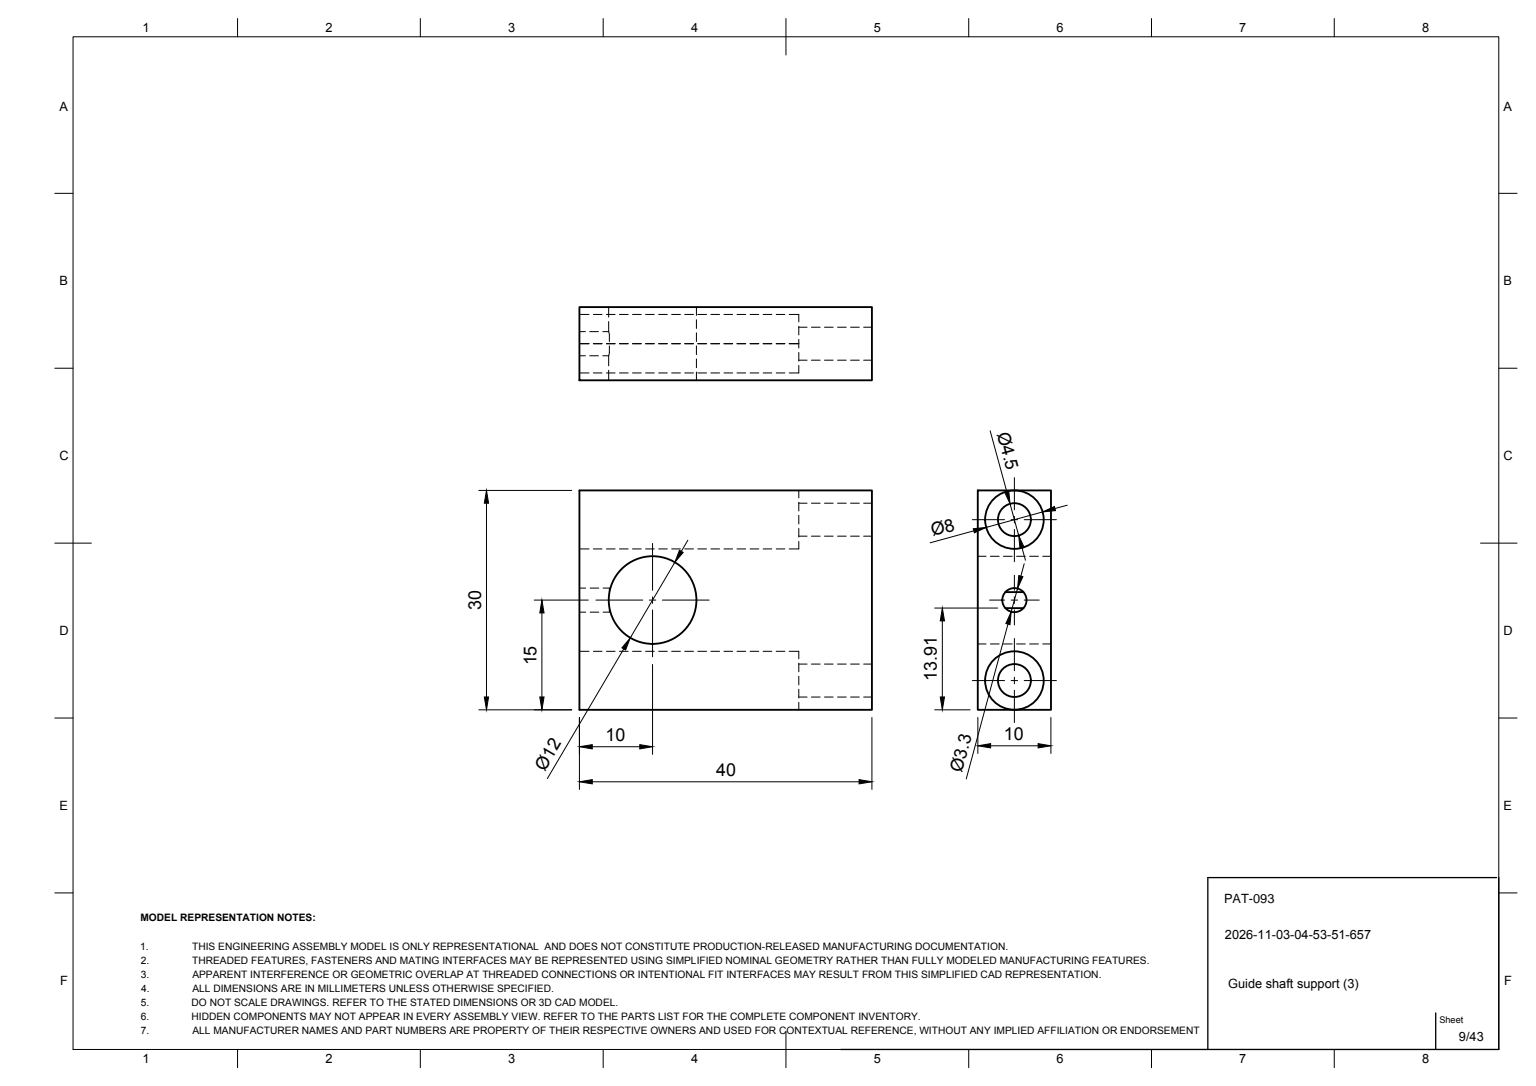
ISO-10303-21;
HEADER;
/* Generated by software containing ST-Developer
 * from STEP Tools, Inc. (www.steptools.com) 
 */

FILE_DESCRIPTION(
/* description */ ('Self-centering screw clamp'),
/* implementation_level */ '2;1');

FILE_NAME(
/* name */ 'Guide shaft support (3).step',
/* time_stamp */ '2026-10-28T03:25:31-07:00',
/* author */ (''),
/* organization */ (''),
/* preprocessor_version */ 'ST-DEVELOPER v20.2',
/* originating_system */ 'Autodesk Translation Framework v15.17.0.0',
/* authorisation */ '');

FILE_SCHEMA (('AUTOMOTIVE_DESIGN { 1 0 10303 214 3 1 1 }'));
ENDSEC;

DATA;
#10=MECHANICAL_DESIGN_GEOMETRIC_PRESENTATION_REPRESENTATION('',(#630),#16799);
#510=B_SPLINE_CURVE_WITH_KNOTS('',3,(#14205,#14206,#14207,#14208,#14209,
#14210),.UNSPECIFIED.,.F.,.F.,(4,2,4),(0.635430324955931,0.687528937234027,
0.750024497760672),.UNSPECIFIED.);
#511=B_SPLINE_CURVE_WITH_KNOTS('',3,(#14214,#14215,#14216,#14217,#14218,
#14219),.UNSPECIFIED.,.F.,.F.,(4,2,4),(0.250008165920224,0.312503726446869,
0.364602338724964),.UNSPECIFIED.);
#512=B_SPLINE_CURVE_WITH_KNOTS('',3,(#14220,#14221,#14222,#14223,#14224,
#14225),.UNSPECIFIED.,.F.,.F.,(4,2,4),(0.135413993115483,0.187512605393579,
0.250008165920224),.UNSPECIFIED.);
#513=B_SPLINE_CURVE_WITH_KNOTS('',3,(#14226,#14227,#14228,#14229,#14230,
#14231),.UNSPECIFIED.,.F.,.F.,(4,2,4),(0.750024497760672,0.812520058287317,
0.864618670565414),.UNSPECIFIED.);
#548=SHAPE_REPRESENTATION_RELATIONSHIP('SRR','None',#17021,#589);
#589=ADVANCED_BREP_SHAPE_REPRESENTATION('',(#678),#16759);
#630=STYLED_ITEM('',(#17326),#678);
#678=MANIFOLD_SOLID_BREP('Body1',#9081);
#763=FACE_BOUND('',#1913,.T.);
#764=FACE_BOUND('',#1916,.T.);
#765=FACE_BOUND('',#1918,.T.);
#766=FACE_BOUND('',#1924,.T.);
#767=FACE_BOUND('',#1927,.T.);
#768=FACE_BOUND('',#1929,.T.);
#769=FACE_BOUND('',#1930,.T.);
#1062=PLANE('',#9751);
#1063=PLANE('',#9756);
#1064=PLANE('',#9760);
#1065=PLANE('',#9765);
#1066=PLANE('',#9767);
#1067=PLANE('',#9775);
#1068=PLANE('',#9776);
#1069=PLANE('',#9777);
#1070=PLANE('',#9778);
#1071=PLANE('',#9779);
#1357=FACE_OUTER_BOUND('',#1906,.T.);
#1358=FACE_OUTER_BOUND('',#1907,.T.);
#1359=FACE_OUTER_BOUND('',#1908,.T.);
#1360=FACE_OUTER_BOUND('',#1909,.T.);
#1361=FACE_OUTER_BOUND('',#1910,.T.);
#1362=FACE_OUTER_BOUND('',#1911,.T.);
#1363=FACE_OUTER_BOUND('',#1912,.T.);
#1364=FACE_OUTER_BOUND('',#1914,.T.);
#1365=FACE_OUTER_BOUND('',#1915,.T.);
#1366=FACE_OUTER_BOUND('',#1917,.T.);
#1367=FACE_OUTER_BOUND('',#1919,.T.);
#1368=FACE_OUTER_BOUND('',#1920,.T.);
#1369=FACE_OUTER_BOUND('',#1921,.T.);
#1370=FACE_OUTER_BOUND('',#1922,.T.);
#1371=FACE_OUTER_BOUND('',#1923,.T.);
#1372=FACE_OUTER_BOUND('',#1925,.T.);
#1373=FACE_OUTER_BOUND('',#1926,.T.);
#1374=FACE_OUTER_BOUND('',#1928,.T.);
#1906=EDGE_LOOP('',(#6535,#6536,#6537,#6538));
#1907=EDGE_LOOP('',(#6539,#6540,#6541,#6542));
#1908=EDGE_LOOP('',(#6543,#6544));
#1909=EDGE_LOOP('',(#6545,#6546,#6547,#6548,#6549,#6550,#6551,#6552,#6553));
#1910=EDGE_LOOP('',(#6554,#6555));
#1911=EDGE_LOOP('',(#6556,#6557,#6558,#6559));
#1912=EDGE_LOOP('',(#6560,#6561));
#1913=EDGE_LOOP('',(#6562));
#1914=EDGE_LOOP('',(#6563,#6564,#6565,#6566));
#1915=EDGE_LOOP('',(#6567,#6568));
#1916=EDGE_LOOP('',(#6569));
#1917=EDGE_LOOP('',(#6570,#6571,#6572,#6573,#6574,#6575,#6576,#6577,#6578,
#6579));
#1918=EDGE_LOOP('',(#6580));
#1919=EDGE_LOOP('',(#6581,#6582,#6583,#6584));
#1920=EDGE_LOOP('',(#6585,#6586,#6587,#6588));
#1921=EDGE_LOOP('',(#6589,#6590,#6591,#6592,#6593,#6594,#6595,#6596,#6597,
#6598,#6599,#6600));
#1922=EDGE_LOOP('',(#6601,#6602,#6603,#6604,#6605,#6606,#6607));
#1923=EDGE_LOOP('',(#6608,#6609,#6610,#6611));
#1924=EDGE_LOOP('',(#6612));
#1925=EDGE_LOOP('',(#6613,#6614,#6615,#6616,#6617,#6618,#6619));
#1926=EDGE_LOOP('',(#6620,#6621,#6622,#6623));
#1927=EDGE_LOOP('',(#6624));
#1928=EDGE_LOOP('',(#6625,#6626,#6627,#6628));
#1929=EDGE_LOOP('',(#6629));
#1930=EDGE_LOOP('',(#6630));
#2706=LINE('',#14182,#3279);
#2707=LINE('',#14186,#3280);
#2708=LINE('',#14191,#3281);
#2709=LINE('',#14195,#3282);
#2710=LINE('',#14200,#3283);
#2711=LINE('',#14233,#3284);
#2712=LINE('',#14236,#3285);
#2713=LINE('',#14239,#3286);
#2714=LINE('',#14246,#3287);
#2715=LINE('',#14254,#3288);
#2716=LINE('',#14255,#3289);
#2717=LINE('',#14257,#3290);
#2718=LINE('',#14259,#3291);
#2719=LINE('',#14260,#3292);
#2720=LINE('',#14261,#3293);
#2721=LINE('',#14265,#3294);
#2722=LINE('',#14269,#3295);
#2723=LINE('',#14273,#3296);
#2724=LINE('',#14275,#3297);
#2725=LINE('',#14280,#3298);
#2726=LINE('',#14281,#3299);
#2727=LINE('',#14282,#3300);
#2728=LINE('',#14285,#3301);
#2729=LINE('',#14286,#3302);
#2730=LINE('',#14289,#3303);
#2731=LINE('',#14290,#3304);
#2732=LINE('',#14292,#3305);
#3279=VECTOR('',#11219,0.4);
#3280=VECTOR('',#11222,1.);
#3281=VECTOR('',#11227,0.4);
#3282=VECTOR('',#11230,1.);
#3283=VECTOR('',#11235,1.);
#3284=VECTOR('',#11242,0.164999999999999);
#3285=VECTOR('',#11247,1.);
#3286=VECTOR('',#11252,1.);
#3287=VECTOR('',#11263,1.);
#3288=VECTOR('',#11272,1.);
#3289=VECTOR('',#11273,1.);
#3290=VECTOR('',#11274,1.);
#3291=VECTOR('',#11275,1.);
#3292=VECTOR('',#11276,1.);
#3293=VECTOR('',#11277,1.);
#3294=VECTOR('',#11282,0.225);
#3295=VECTOR('',#11287,0.225);
#3296=VECTOR('',#11292,0.6);
#3297=VECTOR('',#11293,0.6);
#3298=VECTOR('',#11298,1.);
#3299=VECTOR('',#11299,1.);
#3300=VECTOR('',#11300,1.);
#3301=VECTOR('',#11303,1.);
#3302=VECTOR('',#11304,1.);
#3303=VECTOR('',#11307,1.);
#3304=VECTOR('',#11308,1.);
#3305=VECTOR('',#11311,1.);
#3798=CIRCLE('',#9746,0.4);
#3799=CIRCLE('',#9747,0.4);
#3800=CIRCLE('',#9749,0.4);
#3801=CIRCLE('',#9750,0.4);
#3802=CIRCLE('',#9752,0.164999999999999);
#3803=CIRCLE('',#9754,0.164999999999999);
#3804=CIRCLE('',#9755,0.164999999999999);
#3805=CIRCLE('',#9758,0.4);
#3806=CIRCLE('',#9759,0.4);
#3807=CIRCLE('',#9761,0.225);
#3808=CIRCLE('',#9763,0.4);
#3809=CIRCLE('',#9764,0.4);
#3810=CIRCLE('',#9766,0.225);
#3811=CIRCLE('',#9769,0.225);
#3812=CIRCLE('',#9771,0.225);
#3813=CIRCLE('',#9773,0.6);
#3814=CIRCLE('',#9774,0.6);
#4368=VERTEX_POINT('',#14180);
#4369=VERTEX_POINT('',#14181);
#4370=VERTEX_POINT('',#14183);
#4371=VERTEX_POINT('',#14185);
#4372=VERTEX_POINT('',#14189);
#4373=VERTEX_POINT('',#14190);
#4374=VERTEX_POINT('',#14192);
#4375=VERTEX_POINT('',#14194);
#4376=VERTEX_POINT('',#14198);
#4377=VERTEX_POINT('',#14199);
#4378=VERTEX_POINT('',#14203);
#4379=VERTEX_POINT('',#14204);
#4380=VERTEX_POINT('',#14211);
#4381=VERTEX_POINT('',#14213);
#4382=VERTEX_POINT('',#14232);
#4383=VERTEX_POINT('',#14242);
#4384=VERTEX_POINT('',#14249);
#4385=VERTEX_POINT('',#14252);
#4386=VERTEX_POINT('',#14253);
#4387=VERTEX_POINT('',#14256);
#4388=VERTEX_POINT('',#14258);
#4389=VERTEX_POINT('',#14263);
#4390=VERTEX_POINT('',#14267);
#4391=VERTEX_POINT('',#14271);
#4392=VERTEX_POINT('',#14274);
#4393=VERTEX_POINT('',#14278);
#4394=VERTEX_POINT('',#14279);
#4395=VERTEX_POINT('',#14284);
#4396=VERTEX_POINT('',#14288);
#5192=EDGE_CURVE('',#4368,#4369,#2706,.T.);
#5193=EDGE_CURVE('',#4370,#4368,#3798,.T.);
#5194=EDGE_CURVE('',#4370,#4371,#2707,.T.);
#5195=EDGE_CURVE('',#4369,#4371,#3799,.T.);
#5196=EDGE_CURVE('',#4372,#4373,#2708,.T.);
#5197=EDGE_CURVE('',#4374,#4372,#3800,.T.);
#5198=EDGE_CURVE('',#4374,#4375,#2709,.T.);
#5199=EDGE_CURVE('',#4373,#4375,#3801,.T.);
#5200=EDGE_CURVE('',#4376,#4377,#2710,.T.);
#5201=EDGE_CURVE('',#4376,#4377,#3802,.T.);
#5202=EDGE_CURVE('',#4378,#4379,#510,.T.);
#5203=EDGE_CURVE('',#4380,#4378,#3803,.T.);
#5204=EDGE_CURVE('',#4381,#4380,#511,.T.);
#5205=EDGE_CURVE('',#4377,#4381,#512,.T.);
#5206=EDGE_CURVE('',#4379,#4376,#513,.T.);
#5207=EDGE_CURVE('',#4379,#4382,#2711,.T.);
#5208=EDGE_CURVE('',#4382,#4382,#3804,.T.);
#5209=EDGE_CURVE('',#4380,#4378,#2712,.T.);
#5210=EDGE_CURVE('',#4375,#4373,#3805,.T.);
#5211=EDGE_CURVE('',#4374,#4375,#2713,.T.);
#5212=EDGE_CURVE('',#4372,#4374,#3806,.T.);
#5213=EDGE_CURVE('',#4383,#4383,#3807,.T.);
#5214=EDGE_CURVE('',#4371,#4369,#3808,.T.);
#5215=EDGE_CURVE('',#4370,#4371,#2714,.T.);
#5216=EDGE_CURVE('',#4368,#4370,#3809,.T.);
#5217=EDGE_CURVE('',#4384,#4384,#3810,.T.);
#5218=EDGE_CURVE('',#4385,#4386,#2715,.T.);
#5219=EDGE_CURVE('',#4386,#4375,#2716,.T.);
#5220=EDGE_CURVE('',#4375,#4387,#2717,.T.);
#5221=EDGE_CURVE('',#4387,#4388,#2718,.T.);
#5222=EDGE_CURVE('',#4388,#4371,#2719,.T.);
#5223=EDGE_CURVE('',#4371,#4385,#2720,.T.);
#5224=EDGE_CURVE('',#4389,#4389,#3811,.T.);
#5225=EDGE_CURVE('',#4389,#4383,#2721,.T.);
#5226=EDGE_CURVE('',#4390,#4390,#3812,.T.);
#5227=EDGE_CURVE('',#4390,#4384,#2722,.T.);
#5228=EDGE_CURVE('',#4391,#4391,#3813,.T.);
#5229=EDGE_CURVE('',#4391,#4379,#2723,.T.);
#5230=EDGE_CURVE('',#4381,#4392,#2724,.T.);
#5231=EDGE_CURVE('',#4392,#4392,#3814,.T.);
#5232=EDGE_CURVE('',#4393,#4394,#2725,.T.);
#5233=EDGE_CURVE('',#4394,#4385,#2726,.T.);
#5234=EDGE_CURVE('',#4393,#4388,#2727,.T.);
#5235=EDGE_CURVE('',#4395,#4393,#2728,.T.);
#5236=EDGE_CURVE('',#4395,#4387,#2729,.T.);
#5237=EDGE_CURVE('',#4396,#4395,#2730,.T.);
#5238=EDGE_CURVE('',#4396,#4386,#2731,.T.);
#5239=EDGE_CURVE('',#4394,#4396,#2732,.T.);
#6535=ORIENTED_EDGE('',*,*,#5192,.F.);
#6536=ORIENTED_EDGE('',*,*,#5193,.F.);
#6537=ORIENTED_EDGE('',*,*,#5194,.T.);
#6538=ORIENTED_EDGE('',*,*,#5195,.F.);
#6539=ORIENTED_EDGE('',*,*,#5196,.F.);
#6540=ORIENTED_EDGE('',*,*,#5197,.F.);
#6541=ORIENTED_EDGE('',*,*,#5198,.T.);
#6542=ORIENTED_EDGE('',*,*,#5199,.F.);
#6543=ORIENTED_EDGE('',*,*,#5200,.F.);
#6544=ORIENTED_EDGE('',*,*,#5201,.T.);
#6545=ORIENTED_EDGE('',*,*,#5202,.F.);
#6546=ORIENTED_EDGE('',*,*,#5203,.F.);
#6547=ORIENTED_EDGE('',*,*,#5204,.F.);
#6548=ORIENTED_EDGE('',*,*,#5205,.F.);
#6549=ORIENTED_EDGE('',*,*,#5201,.F.);
#6550=ORIENTED_EDGE('',*,*,#5206,.F.);
#6551=ORIENTED_EDGE('',*,*,#5207,.T.);
#6552=ORIENTED_EDGE('',*,*,#5208,.F.);
#6553=ORIENTED_EDGE('',*,*,#5207,.F.);
#6554=ORIENTED_EDGE('',*,*,#5209,.F.);
#6555=ORIENTED_EDGE('',*,*,#5203,.T.);
#6556=ORIENTED_EDGE('',*,*,#5196,.T.);
#6557=ORIENTED_EDGE('',*,*,#5210,.F.);
#6558=ORIENTED_EDGE('',*,*,#5211,.F.);
#6559=ORIENTED_EDGE('',*,*,#5212,.F.);
#6560=ORIENTED_EDGE('',*,*,#5197,.T.);
#6561=ORIENTED_EDGE('',*,*,#5212,.T.);
#6562=ORIENTED_EDGE('',*,*,#5213,.F.);
#6563=ORIENTED_EDGE('',*,*,#5192,.T.);
#6564=ORIENTED_EDGE('',*,*,#5214,.F.);
#6565=ORIENTED_EDGE('',*,*,#5215,.F.);
#6566=ORIENTED_EDGE('',*,*,#5216,.F.);
#6567=ORIENTED_EDGE('',*,*,#5193,.T.);
#6568=ORIENTED_EDGE('',*,*,#5216,.T.);
#6569=ORIENTED_EDGE('',*,*,#5217,.F.);
#6570=ORIENTED_EDGE('',*,*,#5218,.T.);
#6571=ORIENTED_EDGE('',*,*,#5219,.T.);
#6572=ORIENTED_EDGE('',*,*,#5210,.T.);
#6573=ORIENTED_EDGE('',*,*,#5199,.T.);
#6574=ORIENTED_EDGE('',*,*,#5220,.T.);
#6575=ORIENTED_EDGE('',*,*,#5221,.T.);
#6576=ORIENTED_EDGE('',*,*,#5222,.T.);
#6577=ORIENTED_EDGE('',*,*,#5214,.T.);
#6578=ORIENTED_EDGE('',*,*,#5195,.T.);
#6579=ORIENTED_EDGE('',*,*,#5223,.T.);
#6580=ORIENTED_EDGE('',*,*,#5208,.T.);
#6581=ORIENTED_EDGE('',*,*,#5224,.F.);
#6582=ORIENTED_EDGE('',*,*,#5225,.T.);
#6583=ORIENTED_EDGE('',*,*,#5213,.T.);
#6584=ORIENTED_EDGE('',*,*,#5225,.F.);
#6585=ORIENTED_EDGE('',*,*,#5226,.F.);
#6586=ORIENTED_EDGE('',*,*,#5227,.T.);
#6587=ORIENTED_EDGE('',*,*,#5217,.T.);
#6588=ORIENTED_EDGE('',*,*,#5227,.F.);
#6589=ORIENTED_EDGE('',*,*,#5228,.F.);
#6590=ORIENTED_EDGE('',*,*,#5229,.T.);
#6591=ORIENTED_EDGE('',*,*,#5206,.T.);
#6592=ORIENTED_EDGE('',*,*,#5200,.T.);
#6593=ORIENTED_EDGE('',*,*,#5205,.T.);
#6594=ORIENTED_EDGE('',*,*,#5230,.T.);
#6595=ORIENTED_EDGE('',*,*,#5231,.F.);
#6596=ORIENTED_EDGE('',*,*,#5230,.F.);
#6597=ORIENTED_EDGE('',*,*,#5204,.T.);
#6598=ORIENTED_EDGE('',*,*,#5209,.T.);
#6599=ORIENTED_EDGE('',*,*,#5202,.T.);
#6600=ORIENTED_EDGE('',*,*,#5229,.F.);
#6601=ORIENTED_EDGE('',*,*,#5232,.T.);
#6602=ORIENTED_EDGE('',*,*,#5233,.T.);
#6603=ORIENTED_EDGE('',*,*,#5223,.F.);
#6604=ORIENTED_EDGE('',*,*,#5194,.F.);
#6605=ORIENTED_EDGE('',*,*,#5215,.T.);
#6606=ORIENTED_EDGE('',*,*,#5222,.F.);
#6607=ORIENTED_EDGE('',*,*,#5234,.F.);
#6608=ORIENTED_EDGE('',*,*,#5235,.T.);
#6609=ORIENTED_EDGE('',*,*,#5234,.T.);
#6610=ORIENTED_EDGE('',*,*,#5221,.F.);
#6611=ORIENTED_EDGE('',*,*,#5236,.F.);
#6612=ORIENTED_EDGE('',*,*,#5231,.T.);
#6613=ORIENTED_EDGE('',*,*,#5237,.T.);
#6614=ORIENTED_EDGE('',*,*,#5236,.T.);
#6615=ORIENTED_EDGE('',*,*,#5220,.F.);
#6616=ORIENTED_EDGE('',*,*,#5198,.F.);
#6617=ORIENTED_EDGE('',*,*,#5211,.T.);
#6618=ORIENTED_EDGE('',*,*,#5219,.F.);
#6619=ORIENTED_EDGE('',*,*,#5238,.F.);
#6620=ORIENTED_EDGE('',*,*,#5239,.T.);
#6621=ORIENTED_EDGE('',*,*,#5238,.T.);
#6622=ORIENTED_EDGE('',*,*,#5218,.F.);
#6623=ORIENTED_EDGE('',*,*,#5233,.F.);
#6624=ORIENTED_EDGE('',*,*,#5228,.T.);
#6625=ORIENTED_EDGE('',*,*,#5239,.F.);
#6626=ORIENTED_EDGE('',*,*,#5232,.F.);
#6627=ORIENTED_EDGE('',*,*,#5235,.F.);
#6628=ORIENTED_EDGE('',*,*,#5237,.F.);
#6629=ORIENTED_EDGE('',*,*,#5224,.T.);
#6630=ORIENTED_EDGE('',*,*,#5226,.T.);
#8393=CYLINDRICAL_SURFACE('',#9745,0.4);
#8394=CYLINDRICAL_SURFACE('',#9748,0.4);
#8395=CYLINDRICAL_SURFACE('',#9753,0.164999999999999);
#8396=CYLINDRICAL_SURFACE('',#9757,0.4);
#8397=CYLINDRICAL_SURFACE('',#9762,0.4);
#8398=CYLINDRICAL_SURFACE('',#9768,0.225);
#8399=CYLINDRICAL_SURFACE('',#9770,0.225);
#8400=CYLINDRICAL_SURFACE('',#9772,0.6);
#8655=ADVANCED_FACE('',(#1357),#8393,.F.);
#8656=ADVANCED_FACE('',(#1358),#8394,.F.);
#8657=ADVANCED_FACE('',(#1359),#1062,.T.);
#8658=ADVANCED_FACE('',(#1360),#8395,.F.);
#8659=ADVANCED_FACE('',(#1361),#1063,.T.);
#8660=ADVANCED_FACE('',(#1362),#8396,.F.);
#8661=ADVANCED_FACE('',(#1363,#763),#1064,.T.);
#8662=ADVANCED_FACE('',(#1364),#8397,.F.);
#8663=ADVANCED_FACE('',(#1365,#764),#1065,.T.);
#8664=ADVANCED_FACE('',(#1366,#765),#1066,.T.);
#8665=ADVANCED_FACE('',(#1367),#8398,.F.);
#8666=ADVANCED_FACE('',(#1368),#8399,.F.);
#8667=ADVANCED_FACE('',(#1369),#8400,.F.);
#8668=ADVANCED_FACE('',(#1370),#1067,.T.);
#8669=ADVANCED_FACE('',(#1371,#766),#1068,.T.);
#8670=ADVANCED_FACE('',(#1372),#1069,.T.);
#8671=ADVANCED_FACE('',(#1373,#767),#1070,.T.);
#8672=ADVANCED_FACE('',(#1374,#768,#769),#1071,.F.);
#9081=CLOSED_SHELL('',(#8655,#8656,#8657,#8658,#8659,#8660,#8661,#8662,
#8663,#8664,#8665,#8666,#8667,#8668,#8669,#8670,#8671,#8672));
#9744=AXIS2_PLACEMENT_3D('',#14178,#11215,#11216);
#9745=AXIS2_PLACEMENT_3D('',#14179,#11217,#11218);
#9746=AXIS2_PLACEMENT_3D('',#14184,#11220,#11221);
#9747=AXIS2_PLACEMENT_3D('',#14187,#11223,#11224);
#9748=AXIS2_PLACEMENT_3D('',#14188,#11225,#11226);
#9749=AXIS2_PLACEMENT_3D('',#14193,#11228,#11229);
#9750=AXIS2_PLACEMENT_3D('',#14196,#11231,#11232);
#9751=AXIS2_PLACEMENT_3D('',#14197,#11233,#11234);
#9752=AXIS2_PLACEMENT_3D('',#14201,#11236,#11237);
#9753=AXIS2_PLACEMENT_3D('',#14202,#11238,#11239);
#9754=AXIS2_PLACEMENT_3D('',#14212,#11240,#11241);
#9755=AXIS2_PLACEMENT_3D('',#14234,#11243,#11244);
#9756=AXIS2_PLACEMENT_3D('',#14235,#11245,#11246);
#9757=AXIS2_PLACEMENT_3D('',#14237,#11248,#11249);
#9758=AXIS2_PLACEMENT_3D('',#14238,#11250,#11251);
#9759=AXIS2_PLACEMENT_3D('',#14240,#11253,#11254);
#9760=AXIS2_PLACEMENT_3D('',#14241,#11255,#11256);
#9761=AXIS2_PLACEMENT_3D('',#14243,#11257,#11258);
#9762=AXIS2_PLACEMENT_3D('',#14244,#11259,#11260);
#9763=AXIS2_PLACEMENT_3D('',#14245,#11261,#11262);
#9764=AXIS2_PLACEMENT_3D('',#14247,#11264,#11265);
#9765=AXIS2_PLACEMENT_3D('',#14248,#11266,#11267);
#9766=AXIS2_PLACEMENT_3D('',#14250,#11268,#11269);
#9767=AXIS2_PLACEMENT_3D('',#14251,#11270,#11271);
#9768=AXIS2_PLACEMENT_3D('',#14262,#11278,#11279);
#9769=AXIS2_PLACEMENT_3D('',#14264,#11280,#11281);
#9770=AXIS2_PLACEMENT_3D('',#14266,#11283,#11284);
#9771=AXIS2_PLACEMENT_3D('',#14268,#11285,#11286);
#9772=AXIS2_PLACEMENT_3D('',#14270,#11288,#11289);
#9773=AXIS2_PLACEMENT_3D('',#14272,#11290,#11291);
#9774=AXIS2_PLACEMENT_3D('',#14276,#11294,#11295);
#9775=AXIS2_PLACEMENT_3D('',#14277,#11296,#11297);
#9776=AXIS2_PLACEMENT_3D('',#14283,#11301,#11302);
#9777=AXIS2_PLACEMENT_3D('',#14287,#11305,#11306);
#9778=AXIS2_PLACEMENT_3D('',#14291,#11309,#11310);
#9779=AXIS2_PLACEMENT_3D('',#14293,#11312,#11313);
#11215=DIRECTION('axis',(0.,0.,1.));
#11216=DIRECTION('refdir',(1.,0.,0.));
#11217=DIRECTION('center_axis',(0.,0.,1.));
#11218=DIRECTION('ref_axis',(1.,0.,0.));
#11219=DIRECTION('',(0.,0.,1.));
#11220=DIRECTION('center_axis',(0.,0.,1.));
#11221=DIRECTION('ref_axis',(1.,0.,0.));
#11222=DIRECTION('',(0.,0.,1.));
#11223=DIRECTION('center_axis',(0.,0.,-1.));
#11224=DIRECTION('ref_axis',(1.,0.,0.));
#11225=DIRECTION('center_axis',(0.,0.,1.));
#11226=DIRECTION('ref_axis',(1.,0.,0.));
#11227=DIRECTION('',(0.,0.,1.));
#11228=DIRECTION('center_axis',(0.,0.,1.));
#11229=DIRECTION('ref_axis',(1.,0.,0.));
#11230=DIRECTION('',(0.,0.,1.));
#11231=DIRECTION('center_axis',(0.,0.,-1.));
#11232=DIRECTION('ref_axis',(1.,0.,0.));
#11233=DIRECTION('center_axis',(0.,0.,1.));
#11234=DIRECTION('ref_axis',(1.,0.,0.));
#11235=DIRECTION('',(1.,0.,0.));
#11236=DIRECTION('center_axis',(0.,0.,1.));
#11237=DIRECTION('ref_axis',(1.,0.,0.));
#11238=DIRECTION('center_axis',(0.,0.,1.));
#11239=DIRECTION('ref_axis',(1.,0.,0.));
#11240=DIRECTION('center_axis',(0.,0.,1.));
#11241=DIRECTION('ref_axis',(1.,0.,0.));
#11242=DIRECTION('',(0.,0.,1.));
#11243=DIRECTION('center_axis',(0.,0.,-1.));
#11244=DIRECTION('ref_axis',(1.,0.,0.));
#11245=DIRECTION('center_axis',(0.,0.,1.));
#11246=DIRECTION('ref_axis',(1.,0.,0.));
#11247=DIRECTION('',(-1.,0.,0.));
#11248=DIRECTION('center_axis',(0.,0.,1.));
#11249=DIRECTION('ref_axis',(1.,0.,0.));
#11250=DIRECTION('center_axis',(0.,0.,-1.));
#11251=DIRECTION('ref_axis',(1.,0.,0.));
#11252=DIRECTION('',(0.,0.,1.));
#11253=DIRECTION('center_axis',(0.,0.,1.));
#11254=DIRECTION('ref_axis',(1.,0.,0.));
#11255=DIRECTION('center_axis',(0.,0.,1.));
#11256=DIRECTION('ref_axis',(1.,0.,0.));
#11257=DIRECTION('center_axis',(0.,0.,1.));
#11258=DIRECTION('ref_axis',(1.,0.,0.));
#11259=DIRECTION('center_axis',(0.,0.,1.));
#11260=DIRECTION('ref_axis',(1.,0.,0.));
#11261=DIRECTION('center_axis',(0.,0.,-1.));
#11262=DIRECTION('ref_axis',(1.,0.,0.));
#11263=DIRECTION('',(0.,0.,1.));
#11264=DIRECTION('center_axis',(0.,0.,1.));
#11265=DIRECTION('ref_axis',(1.,0.,0.));
#11266=DIRECTION('center_axis',(0.,0.,1.));
#11267=DIRECTION('ref_axis',(1.,0.,0.));
#11268=DIRECTION('center_axis',(0.,0.,1.));
#11269=DIRECTION('ref_axis',(1.,0.,0.));
#11270=DIRECTION('center_axis',(0.,0.,1.));
#11271=DIRECTION('ref_axis',(1.,0.,0.));
#11272=DIRECTION('',(0.,-1.,0.));
#11273=DIRECTION('',(1.,0.,0.));
#11274=DIRECTION('',(1.,0.,0.));
#11275=DIRECTION('',(0.,1.,0.));
#11276=DIRECTION('',(-1.,0.,0.));
#11277=DIRECTION('',(-1.,0.,0.));
#11278=DIRECTION('center_axis',(0.,0.,1.));
#11279=DIRECTION('ref_axis',(1.,0.,0.));
#11280=DIRECTION('center_axis',(0.,0.,1.));
#11281=DIRECTION('ref_axis',(1.,0.,0.));
#11282=DIRECTION('',(0.,0.,1.));
#11283=DIRECTION('center_axis',(0.,0.,1.));
#11284=DIRECTION('ref_axis',(1.,0.,0.));
#11285=DIRECTION('center_axis',(0.,0.,1.));
#11286=DIRECTION('ref_axis',(1.,0.,0.));
#11287=DIRECTION('',(0.,0.,1.));
#11288=DIRECTION('center_axis',(1.,0.,0.));
#11289=DIRECTION('ref_axis',(0.,0.,-1.));
#11290=DIRECTION('center_axis',(1.,0.,0.));
#11291=DIRECTION('ref_axis',(0.,0.,-1.));
#11292=DIRECTION('',(1.,0.,0.));
#11293=DIRECTION('',(1.,0.,0.));
#11294=DIRECTION('center_axis',(-1.,0.,0.));
#11295=DIRECTION('ref_axis',(0.,0.,-1.));
#11296=DIRECTION('center_axis',(0.,1.,0.));
#11297=DIRECTION('ref_axis',(-1.,0.,0.));
#11298=DIRECTION('',(-1.,0.,0.));
#11299=DIRECTION('',(0.,0.,1.));
#11300=DIRECTION('',(0.,0.,1.));
#11301=DIRECTION('center_axis',(1.,0.,0.));
#11302=DIRECTION('ref_axis',(0.,1.,0.));
#11303=DIRECTION('',(0.,1.,0.));
#11304=DIRECTION('',(0.,0.,1.));
#11305=DIRECTION('center_axis',(0.,-1.,0.));
#11306=DIRECTION('ref_axis',(1.,0.,0.));
#11307=DIRECTION('',(1.,0.,0.));
#11308=DIRECTION('',(0.,0.,1.));
#11309=DIRECTION('center_axis',(-1.,0.,0.));
#11310=DIRECTION('ref_axis',(0.,-1.,0.));
#11311=DIRECTION('',(0.,-1.,0.));
#11312=DIRECTION('center_axis',(0.,0.,1.));
#11313=DIRECTION('ref_axis',(1.,0.,0.));
#14178=CARTESIAN_POINT('',(0.,0.,0.));
#14179=CARTESIAN_POINT('Origin',(13.5,4.1,2.));
#14180=CARTESIAN_POINT('',(13.1,4.1,2.));
#14181=CARTESIAN_POINT('',(13.1,4.1,5.));
#14182=CARTESIAN_POINT('',(13.1,4.1,2.));
#14183=CARTESIAN_POINT('',(13.5,4.5,2.));
#14184=CARTESIAN_POINT('Origin',(13.5,4.1,2.));
#14185=CARTESIAN_POINT('',(13.5,4.5,5.));
#14186=CARTESIAN_POINT('',(13.5,4.5,2.));
#14187=CARTESIAN_POINT('Origin',(13.5,4.1,5.));
#14188=CARTESIAN_POINT('Origin',(13.5,1.9,2.));
#14189=CARTESIAN_POINT('',(13.1,1.9,2.));
#14190=CARTESIAN_POINT('',(13.1,1.9,5.));
#14191=CARTESIAN_POINT('',(13.1,1.9,2.));
#14192=CARTESIAN_POINT('',(13.5,1.5,2.));
#14193=CARTESIAN_POINT('Origin',(13.5,1.9,2.));
#14194=CARTESIAN_POINT('',(13.5,1.5,5.));
#14195=CARTESIAN_POINT('',(13.5,1.5,2.));
#14196=CARTESIAN_POINT('Origin',(13.5,1.9,5.));
#14197=CARTESIAN_POINT('Origin',(13.5,3.,4.59));
#14198=CARTESIAN_POINT('',(13.3762058159686,2.89091287885364,4.59));
#14199=CARTESIAN_POINT('',(13.6237941840314,2.89091287885364,4.59));
#14200=CARTESIAN_POINT('',(12.9,2.89091287885364,4.59));
#14201=CARTESIAN_POINT('Origin',(13.5,3.,4.59));
#14202=CARTESIAN_POINT('Origin',(13.5,3.,4.59));
#14203=CARTESIAN_POINT('',(13.3762058159686,3.10908712114636,4.59));
#14204=CARTESIAN_POINT('',(13.335,3.,4.6));
#14205=CARTESIAN_POINT('Ctrl Pts',(13.3762058159686,3.10908712114636,4.59));
#14206=CARTESIAN_POINT('Ctrl Pts',(13.3646008648105,3.09591759715261,4.59243495840567));
#14207=CARTESIAN_POINT('Ctrl Pts',(13.3546543563418,3.08022344943772,4.59485638705045));
#14208=CARTESIAN_POINT('Ctrl Pts',(13.339185135366,3.04298016596019,4.59880705606552));
#14209=CARTESIAN_POINT('Ctrl Pts',(13.335,3.02083185350888,4.6));
#14210=CARTESIAN_POINT('Ctrl Pts',(13.335,3.,4.6));
#14211=CARTESIAN_POINT('',(13.6237941840314,3.10908712114636,4.59));
#14212=CARTESIAN_POINT('Origin',(13.5,3.,4.59));
#14213=CARTESIAN_POINT('',(13.665,3.,4.6));
#14214=CARTESIAN_POINT('Ctrl Pts',(13.665,3.,4.6));
#14215=CARTESIAN_POINT('Ctrl Pts',(13.665,3.02083185350888,4.6));
#14216=CARTESIAN_POINT('Ctrl Pts',(13.660814864634,3.04298016596019,4.59880705606552));
#14217=CARTESIAN_POINT('Ctrl Pts',(13.6453456436582,3.08022344943772,4.59485638705045));
#14218=CARTESIAN_POINT('Ctrl Pts',(13.6353991351895,3.09591759715261,4.59243495840567));
#14219=CARTESIAN_POINT('Ctrl Pts',(13.6237941840314,3.10908712114636,4.59));
#14220=CARTESIAN_POINT('Ctrl Pts',(13.6237941840314,2.89091287885364,4.59));
#14221=CARTESIAN_POINT('Ctrl Pts',(13.6353991351895,2.90408240284739,4.59243495840567));
#14222=CARTESIAN_POINT('Ctrl Pts',(13.6453456436582,2.91977655056228,4.59485638705045));
#14223=CARTESIAN_POINT('Ctrl Pts',(13.660814864634,2.95701983403981,4.59880705606552));
#14224=CARTESIAN_POINT('Ctrl Pts',(13.665,2.97916814649112,4.6));
#14225=CARTESIAN_POINT('Ctrl Pts',(13.665,3.,4.6));
#14226=CARTESIAN_POINT('Ctrl Pts',(13.335,3.,4.6));
#14227=CARTESIAN_POINT('Ctrl Pts',(13.335,2.97916814649112,4.6));
#14228=CARTESIAN_POINT('Ctrl Pts',(13.339185135366,2.95701983403981,4.59880705606552));
#14229=CARTESIAN_POINT('Ctrl Pts',(13.3546543563418,2.91977655056228,4.59485638705045));
#14230=CARTESIAN_POINT('Ctrl Pts',(13.3646008648105,2.90408240284739,4.59243495840567));
#14231=CARTESIAN_POINT('Ctrl Pts',(13.3762058159686,2.89091287885364,4.59));
#14232=CARTESIAN_POINT('',(13.335,3.,5.));
#14233=CARTESIAN_POINT('',(13.335,3.,4.59));
#14234=CARTESIAN_POINT('Origin',(13.5,3.,5.));
#14235=CARTESIAN_POINT('Origin',(13.5,3.,4.59));
#14236=CARTESIAN_POINT('',(12.9,3.10908712114636,4.59));
#14237=CARTESIAN_POINT('Origin',(13.5,1.9,2.));
#14238=CARTESIAN_POINT('Origin',(13.5,1.9,5.));
#14239=CARTESIAN_POINT('',(13.5,1.5,2.));
#14240=CARTESIAN_POINT('Origin',(13.5,1.9,2.));
#14241=CARTESIAN_POINT('Origin',(13.5,1.9,2.));
#14242=CARTESIAN_POINT('',(13.275,1.9,2.));
#14243=CARTESIAN_POINT('Origin',(13.5,1.9,2.));
#14244=CARTESIAN_POINT('Origin',(13.5,4.1,2.));
#14245=CARTESIAN_POINT('Origin',(13.5,4.1,5.));
#14246=CARTESIAN_POINT('',(13.5,4.5,2.));
#14247=CARTESIAN_POINT('Origin',(13.5,4.1,2.));
#14248=CARTESIAN_POINT('Origin',(13.5,4.1,2.));
#14249=CARTESIAN_POINT('',(13.275,4.1,2.));
#14250=CARTESIAN_POINT('Origin',(13.5,4.1,2.));
#14251=CARTESIAN_POINT('Origin',(13.5,3.,5.));
#14252=CARTESIAN_POINT('',(13.,4.5,5.));
#14253=CARTESIAN_POINT('',(13.,1.5,5.));
#14254=CARTESIAN_POINT('',(13.,4.5,5.));
#14255=CARTESIAN_POINT('',(13.,1.5,5.));
#14256=CARTESIAN_POINT('',(14.,1.5,5.));
#14257=CARTESIAN_POINT('',(13.,1.5,5.));
#14258=CARTESIAN_POINT('',(14.,4.5,5.));
#14259=CARTESIAN_POINT('',(14.,1.5,5.));
#14260=CARTESIAN_POINT('',(14.,4.5,5.));
#14261=CARTESIAN_POINT('',(14.,4.5,5.));
#14262=CARTESIAN_POINT('Origin',(13.5,1.9,0.9));
#14263=CARTESIAN_POINT('',(13.275,1.9,1.));
#14264=CARTESIAN_POINT('Origin',(13.5,1.9,1.));
#14265=CARTESIAN_POINT('',(13.275,1.9,0.9));
#14266=CARTESIAN_POINT('Origin',(13.5,4.1,0.9));
#14267=CARTESIAN_POINT('',(13.275,4.1,1.));
#14268=CARTESIAN_POINT('Origin',(13.5,4.1,1.));
#14269=CARTESIAN_POINT('',(13.275,4.1,0.9));
#14270=CARTESIAN_POINT('Origin',(12.9,3.,4.));
#14271=CARTESIAN_POINT('',(13.,3.,4.6));
#14272=CARTESIAN_POINT('Origin',(13.,3.,4.));
#14273=CARTESIAN_POINT('',(12.9,3.,4.6));
#14274=CARTESIAN_POINT('',(14.,3.,4.6));
#14275=CARTESIAN_POINT('',(12.9,3.,4.6));
#14276=CARTESIAN_POINT('Origin',(14.,3.,4.));
#14277=CARTESIAN_POINT('Origin',(14.,4.5,1.));
#14278=CARTESIAN_POINT('',(14.,4.5,1.));
#14279=CARTESIAN_POINT('',(13.,4.5,1.));
#14280=CARTESIAN_POINT('',(14.,4.5,1.));
#14281=CARTESIAN_POINT('',(13.,4.5,1.));
#14282=CARTESIAN_POINT('',(14.,4.5,1.));
#14283=CARTESIAN_POINT('Origin',(14.,1.5,1.));
#14284=CARTESIAN_POINT('',(14.,1.5,1.));
#14285=CARTESIAN_POINT('',(14.,1.5,1.));
#14286=CARTESIAN_POINT('',(14.,1.5,1.));
#14287=CARTESIAN_POINT('Origin',(13.,1.5,1.));
#14288=CARTESIAN_POINT('',(13.,1.5,1.));
#14289=CARTESIAN_POINT('',(13.,1.5,1.));
#14290=CARTESIAN_POINT('',(13.,1.5,1.));
#14291=CARTESIAN_POINT('Origin',(13.,4.5,1.));
#14292=CARTESIAN_POINT('',(13.,4.5,1.));
#14293=CARTESIAN_POINT('Origin',(13.5,3.,1.));
#16710=UNCERTAINTY_MEASURE_WITH_UNIT(LENGTH_MEASURE(0.001),#16800,
'DISTANCE_ACCURACY_VALUE',
'Maximum model space distance between geometric entities at asserted c
onnectivities');
#16750=UNCERTAINTY_MEASURE_WITH_UNIT(LENGTH_MEASURE(0.001),#16800,
'DISTANCE_ACCURACY_VALUE',
'Maximum model space distance between geometric entities at asserted c
onnectivities');
#16759=(
GEOMETRIC_REPRESENTATION_CONTEXT(3)
GLOBAL_UNCERTAINTY_ASSIGNED_CONTEXT((#16710))
GLOBAL_UNIT_ASSIGNED_CONTEXT((#16800,#16802,#16803))
REPRESENTATION_CONTEXT('','3D')
);
#16799=(
GEOMETRIC_REPRESENTATION_CONTEXT(3)
GLOBAL_UNCERTAINTY_ASSIGNED_CONTEXT((#16750))
GLOBAL_UNIT_ASSIGNED_CONTEXT((#16800,#16802,#16803))
REPRESENTATION_CONTEXT('','3D')
);
#16800=(
LENGTH_UNIT()
NAMED_UNIT(*)
SI_UNIT(.CENTI.,.METRE.)
);
#16802=(
NAMED_UNIT(*)
PLANE_ANGLE_UNIT()
SI_UNIT($,.RADIAN.)
);
#16803=(
NAMED_UNIT(*)
SI_UNIT($,.STERADIAN.)
SOLID_ANGLE_UNIT()
);
#16812=SHAPE_DEFINITION_REPRESENTATION(#16860,#17021);
#16860=PRODUCT_DEFINITION_SHAPE('',$,#17070);
#17021=SHAPE_REPRESENTATION('',(#9744),#16759);
#17061=PRODUCT_DEFINITION_CONTEXT('part definition',#17207,'design');
#17070=PRODUCT_DEFINITION('Guide shaft support (3)',
'Guide shaft support (3)',#17118,#17061);
#17118=PRODUCT_DEFINITION_FORMATION('',$,#17217);
#17207=APPLICATION_CONTEXT(
'Core Data for Automotive Mechanical Design Process');
#17208=PRODUCT_CONTEXT('part definition',#17207,'mechanical');
#17217=PRODUCT('Guide shaft support (3)','Guide shaft support (3)',
'Guide shaft support (3)',(#17208));
#17320=COLOUR_RGB('Grey',0.48,0.52,0.57);
#17321=FILL_AREA_STYLE_COLOUR('',#17320);
#17322=FILL_AREA_STYLE('',(#17321));
#17323=SURFACE_STYLE_FILL_AREA(#17322);
#17324=SURFACE_SIDE_STYLE('',(#17323));
#17325=SURFACE_STYLE_USAGE(.BOTH.,#17324);
#17326=PRESENTATION_STYLE_ASSIGNMENT((#17325));
ENDSEC;
END-ISO-10303-21;
